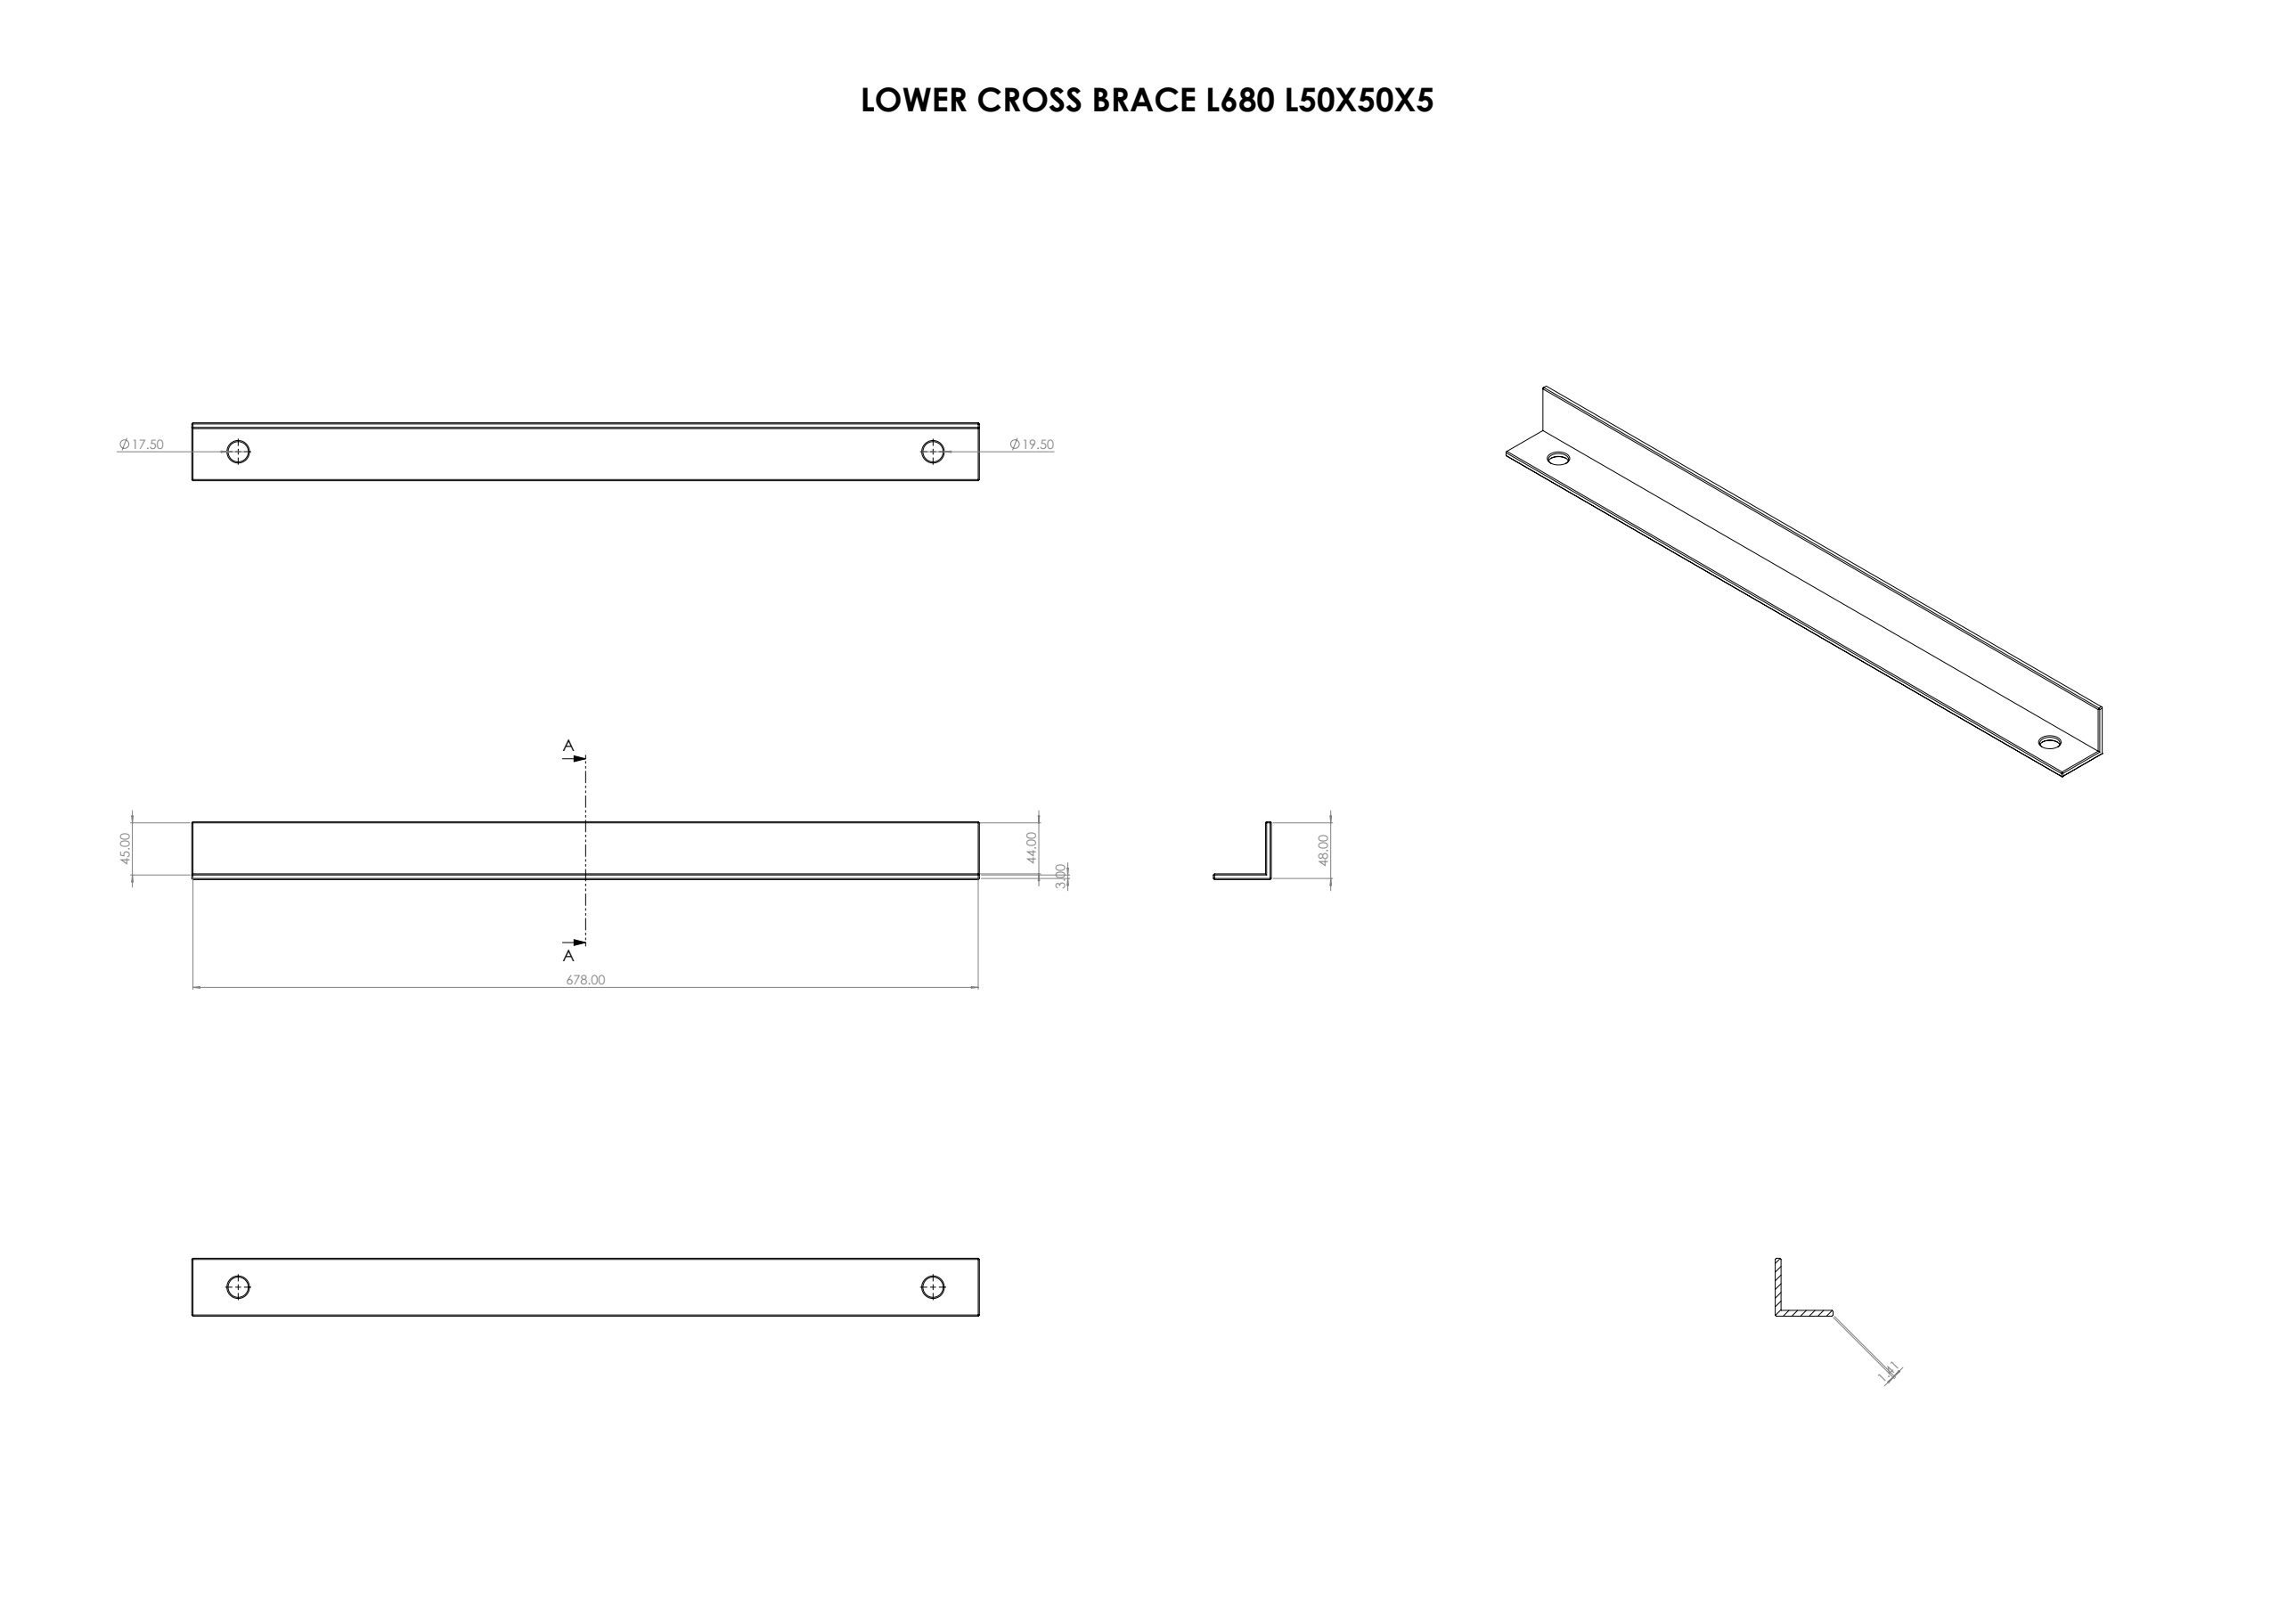
ISO-10303-21;
HEADER;
/* Generated by software containing ST-Developer
 * from STEP Tools, Inc. (www.steptools.com) 
 */

FILE_DESCRIPTION(
/* description */ (''),
/* implementation_level */ '2;1');

FILE_NAME(
/* name */ '08_Lower_Cross_Brace_L680_L50x50x5.step',
/* time_stamp */ '2026-10-20T10:03:03-07:00',
/* author */ (''),
/* organization */ (''),
/* preprocessor_version */ 'ST-DEVELOPER v20.2',
/* originating_system */ 'Autodesk Translation Framework v15.15.0.0',
/* authorisation */ '');

FILE_SCHEMA (('AUTOMOTIVE_DESIGN { 1 0 10303 214 3 1 1 }'));
ENDSEC;

DATA;
#10=MECHANICAL_DESIGN_GEOMETRIC_PRESENTATION_REPRESENTATION('',(#527),#71492);
#385=SHAPE_REPRESENTATION_RELATIONSHIP('SRR','None',#71606,#404);
#404=ADVANCED_BREP_SHAPE_REPRESENTATION('',(#423),#71476);
#423=MANIFOLD_SOLID_BREP('Brace',#28462);
#527=STYLED_ITEM('',(#71873),#423);
#1573=CYLINDRICAL_SURFACE('',#29328,0.875);
#1574=CYLINDRICAL_SURFACE('',#29333,0.875);
#1914=FACE_BOUND('',#5135,.T.);
#1915=FACE_BOUND('',#5136,.T.);
#1916=FACE_BOUND('',#5140,.T.);
#1917=FACE_BOUND('',#5141,.T.);
#2230=CIRCLE('',#29316,0.975000000000001);
#2231=CIRCLE('',#29317,0.975000000000001);
#2232=CIRCLE('',#29321,0.975000000000001);
#2233=CIRCLE('',#29322,0.975000000000001);
#2234=CIRCLE('',#29327,0.875);
#2235=CIRCLE('',#29329,0.875);
#2236=CIRCLE('',#29332,0.875);
#2237=CIRCLE('',#29334,0.875);
#2815=CONICAL_SURFACE('',#29326,0.925000000000001,0.785398163397457);
#2816=CONICAL_SURFACE('',#29330,0.925000000000001,0.785398163397457);
#2817=CONICAL_SURFACE('',#29331,0.925000000000001,0.785398163397457);
#2818=CONICAL_SURFACE('',#29335,0.925000000000001,0.785398163397457);
#3506=FACE_OUTER_BOUND('',#5126,.T.);
#3507=FACE_OUTER_BOUND('',#5127,.T.);
#3508=FACE_OUTER_BOUND('',#5128,.T.);
#3509=FACE_OUTER_BOUND('',#5129,.T.);
#3510=FACE_OUTER_BOUND('',#5130,.T.);
#3511=FACE_OUTER_BOUND('',#5131,.T.);
#3512=FACE_OUTER_BOUND('',#5132,.T.);
#3513=FACE_OUTER_BOUND('',#5133,.T.);
#3514=FACE_OUTER_BOUND('',#5134,.T.);
#3515=FACE_OUTER_BOUND('',#5137,.T.);
#3516=FACE_OUTER_BOUND('',#5138,.T.);
#3517=FACE_OUTER_BOUND('',#5139,.T.);
#3518=FACE_OUTER_BOUND('',#5142,.T.);
#3519=FACE_OUTER_BOUND('',#5143,.T.);
#3520=FACE_OUTER_BOUND('',#5144,.T.);
#3521=FACE_OUTER_BOUND('',#5145,.T.);
#3522=FACE_OUTER_BOUND('',#5146,.T.);
#3523=FACE_OUTER_BOUND('',#5147,.T.);
#3524=FACE_OUTER_BOUND('',#5148,.T.);
#3525=FACE_OUTER_BOUND('',#5149,.T.);
#3526=FACE_OUTER_BOUND('',#5150,.T.);
#3527=FACE_OUTER_BOUND('',#5151,.T.);
#3528=FACE_OUTER_BOUND('',#5152,.T.);
#3529=FACE_OUTER_BOUND('',#5153,.T.);
#3530=FACE_OUTER_BOUND('',#5154,.T.);
#3531=FACE_OUTER_BOUND('',#5155,.T.);
#3532=FACE_OUTER_BOUND('',#5156,.T.);
#3533=FACE_OUTER_BOUND('',#5157,.T.);
#3534=FACE_OUTER_BOUND('',#5158,.T.);
#3535=FACE_OUTER_BOUND('',#5159,.T.);
#3536=FACE_OUTER_BOUND('',#5160,.T.);
#5126=EDGE_LOOP('',(#20811,#20812,#20813,#20814,#20815,#20816));
#5127=EDGE_LOOP('',(#20817,#20818,#20819,#20820,#20821,#20822));
#5128=EDGE_LOOP('',(#20823,#20824,#20825,#20826));
#5129=EDGE_LOOP('',(#20827,#20828,#20829,#20830,#20831,#20832));
#5130=EDGE_LOOP('',(#20833,#20834,#20835,#20836,#20837,#20838));
#5131=EDGE_LOOP('',(#20839,#20840,#20841,#20842,#20843,#20844));
#5132=EDGE_LOOP('',(#20845,#20846,#20847,#20848,#20849,#20850));
#5133=EDGE_LOOP('',(#20851,#20852,#20853,#20854,#20855));
#5134=EDGE_LOOP('',(#20856,#20857,#20858,#20859));
#5135=EDGE_LOOP('',(#20860));
#5136=EDGE_LOOP('',(#20861));
#5137=EDGE_LOOP('',(#20862,#20863,#20864,#20865,#20866,#20867));
#5138=EDGE_LOOP('',(#20868,#20869,#20870,#20871,#20872,#20873));
#5139=EDGE_LOOP('',(#20874,#20875,#20876,#20877));
#5140=EDGE_LOOP('',(#20878));
#5141=EDGE_LOOP('',(#20879));
#5142=EDGE_LOOP('',(#20880,#20881,#20882,#20883,#20884,#20885));
#5143=EDGE_LOOP('',(#20886,#20887,#20888,#20889,#20890,#20891));
#5144=EDGE_LOOP('',(#20892,#20893,#20894,#20895,#20896,#20897));
#5145=EDGE_LOOP('',(#20898,#20899,#20900,#20901));
#5146=EDGE_LOOP('',(#20902,#20903,#20904,#20905));
#5147=EDGE_LOOP('',(#20906,#20907,#20908,#20909));
#5148=EDGE_LOOP('',(#20910,#20911,#20912,#20913));
#5149=EDGE_LOOP('',(#20914,#20915,#20916,#20917));
#5150=EDGE_LOOP('',(#20918,#20919,#20920,#20921));
#5151=EDGE_LOOP('',(#20922,#20923,#20924,#20925,#20926));
#5152=EDGE_LOOP('',(#20927,#20928,#20929,#20930,#20931));
#5153=EDGE_LOOP('',(#20932,#20933,#20934,#20935,#20936,#20937));
#5154=EDGE_LOOP('',(#20938,#20939,#20940,#20941));
#5155=EDGE_LOOP('',(#20942,#20943,#20944,#20945,#20946,#20947));
#5156=EDGE_LOOP('',(#20948,#20949,#20950,#20951,#20952,#20953));
#5157=EDGE_LOOP('',(#20954,#20955,#20956,#20957,#20958));
#5158=EDGE_LOOP('',(#20959,#20960,#20961,#20962));
#5159=EDGE_LOOP('',(#20963,#20964,#20965,#20966,#20967,#20968));
#5160=EDGE_LOOP('',(#20969,#20970,#20971,#20972));
#7329=LINE('',#43368,#9817);
#7330=LINE('',#43370,#9818);
#7331=LINE('',#43372,#9819);
#7332=LINE('',#43374,#9820);
#7333=LINE('',#43376,#9821);
#7334=LINE('',#43377,#9822);
#7335=LINE('',#43380,#9823);
#7336=LINE('',#43382,#9824);
#7337=LINE('',#43384,#9825);
#7338=LINE('',#43386,#9826);
#7339=LINE('',#43387,#9827);
#7340=LINE('',#43390,#9828);
#7341=LINE('',#43391,#9829);
#7342=LINE('',#43394,#9830);
#7343=LINE('',#43396,#9831);
#7344=LINE('',#43398,#9832);
#7345=LINE('',#43399,#9833);
#7346=LINE('',#43402,#9834);
#7347=LINE('',#43404,#9835);
#7348=LINE('',#43405,#9836);
#7349=LINE('',#43409,#9837);
#7350=LINE('',#43411,#9838);
#7351=LINE('',#43413,#9839);
#7352=LINE('',#43415,#9840);
#7353=LINE('',#43417,#9841);
#7354=LINE('',#43418,#9842);
#7355=LINE('',#43421,#9843);
#7356=LINE('',#43423,#9844);
#7357=LINE('',#43425,#9845);
#7358=LINE('',#43427,#9846);
#7359=LINE('',#43428,#9847);
#7360=LINE('',#43431,#9848);
#7361=LINE('',#43433,#9849);
#7362=LINE('',#43434,#9850);
#7363=LINE('',#43437,#9851);
#7364=LINE('',#43438,#9852);
#7365=LINE('',#43446,#9853);
#7366=LINE('',#43448,#9854);
#7367=LINE('',#43450,#9855);
#7368=LINE('',#43452,#9856);
#7369=LINE('',#43454,#9857);
#7370=LINE('',#43455,#9858);
#7371=LINE('',#43458,#9859);
#7372=LINE('',#43459,#9860);
#7373=LINE('',#43461,#9861);
#7374=LINE('',#43462,#9862);
#7375=LINE('',#43465,#9863);
#7376=LINE('',#43466,#9864);
#7377=LINE('',#43473,#9865);
#7378=LINE('',#43475,#9866);
#7379=LINE('',#43477,#9867);
#7380=LINE('',#43478,#9868);
#7381=LINE('',#43481,#9869);
#7382=LINE('',#43482,#9870);
#7383=LINE('',#43484,#9871);
#7384=LINE('',#43486,#9872);
#7385=LINE('',#43487,#9873);
#7386=LINE('',#43490,#9874);
#7387=LINE('',#43495,#9875);
#7388=LINE('',#43497,#9876);
#7389=LINE('',#43500,#9877);
#7390=LINE('',#43505,#9878);
#7391=LINE('',#43507,#9879);
#7392=LINE('',#43510,#9880);
#7393=LINE('',#43511,#9881);
#7394=LINE('',#43513,#9882);
#7395=LINE('',#43514,#9883);
#7396=LINE('',#43516,#9884);
#7397=LINE('',#43517,#9885);
#7398=LINE('',#43521,#9886);
#7399=LINE('',#43522,#9887);
#7400=LINE('',#43524,#9888);
#7401=LINE('',#43525,#9889);
#9817=VECTOR('',#33122,1.);
#9818=VECTOR('',#33123,1.);
#9819=VECTOR('',#33124,1.);
#9820=VECTOR('',#33125,1.);
#9821=VECTOR('',#33126,1.);
#9822=VECTOR('',#33127,1.);
#9823=VECTOR('',#33130,1.);
#9824=VECTOR('',#33131,1.);
#9825=VECTOR('',#33132,1.);
#9826=VECTOR('',#33133,1.);
#9827=VECTOR('',#33134,1.);
#9828=VECTOR('',#33137,1.);
#9829=VECTOR('',#33138,1.);
#9830=VECTOR('',#33141,1.);
#9831=VECTOR('',#33142,1.);
#9832=VECTOR('',#33143,1.);
#9833=VECTOR('',#33144,1.);
#9834=VECTOR('',#33147,1.);
#9835=VECTOR('',#33148,1.);
#9836=VECTOR('',#33149,1.);
#9837=VECTOR('',#33152,1.);
#9838=VECTOR('',#33153,1.);
#9839=VECTOR('',#33154,1.);
#9840=VECTOR('',#33155,1.);
#9841=VECTOR('',#33156,1.);
#9842=VECTOR('',#33157,1.);
#9843=VECTOR('',#33160,1.);
#9844=VECTOR('',#33161,1.);
#9845=VECTOR('',#33162,1.);
#9846=VECTOR('',#33163,1.);
#9847=VECTOR('',#33164,1.);
#9848=VECTOR('',#33167,1.);
#9849=VECTOR('',#33168,1.);
#9850=VECTOR('',#33169,1.);
#9851=VECTOR('',#33172,1.);
#9852=VECTOR('',#33173,1.);
#9853=VECTOR('',#33180,1.);
#9854=VECTOR('',#33181,1.);
#9855=VECTOR('',#33182,1.);
#9856=VECTOR('',#33183,1.);
#9857=VECTOR('',#33184,1.);
#9858=VECTOR('',#33185,1.);
#9859=VECTOR('',#33188,1.);
#9860=VECTOR('',#33189,1.);
#9861=VECTOR('',#33190,1.);
#9862=VECTOR('',#33191,1.);
#9863=VECTOR('',#33194,1.);
#9864=VECTOR('',#33195,1.);
#9865=VECTOR('',#33202,1.);
#9866=VECTOR('',#33203,1.);
#9867=VECTOR('',#33204,1.);
#9868=VECTOR('',#33205,1.);
#9869=VECTOR('',#33208,1.);
#9870=VECTOR('',#33209,1.);
#9871=VECTOR('',#33212,1.);
#9872=VECTOR('',#33213,1.);
#9873=VECTOR('',#33214,1.);
#9874=VECTOR('',#33217,0.925000000000001);
#9875=VECTOR('',#33224,0.875);
#9876=VECTOR('',#33227,0.925000000000001);
#9877=VECTOR('',#33230,0.925000000000001);
#9878=VECTOR('',#33237,0.875);
#9879=VECTOR('',#33240,0.925000000000001);
#9880=VECTOR('',#33243,1.);
#9881=VECTOR('',#33244,1.);
#9882=VECTOR('',#33247,1.);
#9883=VECTOR('',#33248,1.);
#9884=VECTOR('',#33251,1.);
#9885=VECTOR('',#33252,1.);
#9886=VECTOR('',#33259,1.);
#9887=VECTOR('',#33260,1.);
#9888=VECTOR('',#33263,1.);
#9889=VECTOR('',#33264,1.);
#12183=VERTEX_POINT('',#43366);
#12184=VERTEX_POINT('',#43367);
#12185=VERTEX_POINT('',#43369);
#12186=VERTEX_POINT('',#43371);
#12187=VERTEX_POINT('',#43373);
#12188=VERTEX_POINT('',#43375);
#12189=VERTEX_POINT('',#43379);
#12190=VERTEX_POINT('',#43381);
#12191=VERTEX_POINT('',#43383);
#12192=VERTEX_POINT('',#43385);
#12193=VERTEX_POINT('',#43389);
#12194=VERTEX_POINT('',#43393);
#12195=VERTEX_POINT('',#43395);
#12196=VERTEX_POINT('',#43397);
#12197=VERTEX_POINT('',#43401);
#12198=VERTEX_POINT('',#43403);
#12199=VERTEX_POINT('',#43407);
#12200=VERTEX_POINT('',#43408);
#12201=VERTEX_POINT('',#43410);
#12202=VERTEX_POINT('',#43412);
#12203=VERTEX_POINT('',#43414);
#12204=VERTEX_POINT('',#43416);
#12205=VERTEX_POINT('',#43420);
#12206=VERTEX_POINT('',#43422);
#12207=VERTEX_POINT('',#43424);
#12208=VERTEX_POINT('',#43426);
#12209=VERTEX_POINT('',#43430);
#12210=VERTEX_POINT('',#43432);
#12211=VERTEX_POINT('',#43436);
#12212=VERTEX_POINT('',#43439);
#12213=VERTEX_POINT('',#43441);
#12214=VERTEX_POINT('',#43444);
#12215=VERTEX_POINT('',#43445);
#12216=VERTEX_POINT('',#43447);
#12217=VERTEX_POINT('',#43449);
#12218=VERTEX_POINT('',#43451);
#12219=VERTEX_POINT('',#43453);
#12220=VERTEX_POINT('',#43457);
#12221=VERTEX_POINT('',#43460);
#12222=VERTEX_POINT('',#43464);
#12223=VERTEX_POINT('',#43467);
#12224=VERTEX_POINT('',#43469);
#12225=VERTEX_POINT('',#43472);
#12226=VERTEX_POINT('',#43474);
#12227=VERTEX_POINT('',#43476);
#12228=VERTEX_POINT('',#43480);
#12229=VERTEX_POINT('',#43485);
#12230=VERTEX_POINT('',#43489);
#12231=VERTEX_POINT('',#43493);
#12232=VERTEX_POINT('',#43499);
#12233=VERTEX_POINT('',#43503);
#12234=VERTEX_POINT('',#43509);
#15289=EDGE_CURVE('',#12183,#12184,#7329,.T.);
#15290=EDGE_CURVE('',#12184,#12185,#7330,.T.);
#15291=EDGE_CURVE('',#12185,#12186,#7331,.T.);
#15292=EDGE_CURVE('',#12186,#12187,#7332,.T.);
#15293=EDGE_CURVE('',#12187,#12188,#7333,.T.);
#15294=EDGE_CURVE('',#12188,#12183,#7334,.T.);
#15295=EDGE_CURVE('',#12185,#12189,#7335,.T.);
#15296=EDGE_CURVE('',#12190,#12189,#7336,.T.);
#15297=EDGE_CURVE('',#12190,#12191,#7337,.T.);
#15298=EDGE_CURVE('',#12191,#12192,#7338,.T.);
#15299=EDGE_CURVE('',#12192,#12186,#7339,.T.);
#15300=EDGE_CURVE('',#12193,#12184,#7340,.T.);
#15301=EDGE_CURVE('',#12189,#12193,#7341,.T.);
#15302=EDGE_CURVE('',#12194,#12183,#7342,.T.);
#15303=EDGE_CURVE('',#12194,#12195,#7343,.T.);
#15304=EDGE_CURVE('',#12195,#12196,#7344,.T.);
#15305=EDGE_CURVE('',#12193,#12196,#7345,.T.);
#15306=EDGE_CURVE('',#12196,#12197,#7346,.T.);
#15307=EDGE_CURVE('',#12197,#12198,#7347,.T.);
#15308=EDGE_CURVE('',#12198,#12190,#7348,.T.);
#15309=EDGE_CURVE('',#12199,#12200,#7349,.T.);
#15310=EDGE_CURVE('',#12200,#12201,#7350,.T.);
#15311=EDGE_CURVE('',#12201,#12202,#7351,.T.);
#15312=EDGE_CURVE('',#12202,#12203,#7352,.T.);
#15313=EDGE_CURVE('',#12203,#12204,#7353,.T.);
#15314=EDGE_CURVE('',#12204,#12199,#7354,.T.);
#15315=EDGE_CURVE('',#12205,#12202,#7355,.T.);
#15316=EDGE_CURVE('',#12205,#12206,#7356,.T.);
#15317=EDGE_CURVE('',#12206,#12207,#7357,.T.);
#15318=EDGE_CURVE('',#12208,#12207,#7358,.T.);
#15319=EDGE_CURVE('',#12208,#12203,#7359,.T.);
#15320=EDGE_CURVE('',#12201,#12209,#7360,.T.);
#15321=EDGE_CURVE('',#12210,#12209,#7361,.T.);
#15322=EDGE_CURVE('',#12210,#12205,#7362,.T.);
#15323=EDGE_CURVE('',#12211,#12200,#7363,.T.);
#15324=EDGE_CURVE('',#12209,#12211,#7364,.T.);
#15325=EDGE_CURVE('',#12212,#12212,#2230,.T.);
#15326=EDGE_CURVE('',#12213,#12213,#2231,.T.);
#15327=EDGE_CURVE('',#12214,#12215,#7365,.T.);
#15328=EDGE_CURVE('',#12215,#12216,#7366,.T.);
#15329=EDGE_CURVE('',#12216,#12217,#7367,.T.);
#15330=EDGE_CURVE('',#12217,#12218,#7368,.T.);
#15331=EDGE_CURVE('',#12218,#12219,#7369,.T.);
#15332=EDGE_CURVE('',#12219,#12214,#7370,.T.);
#15333=EDGE_CURVE('',#12216,#12220,#7371,.T.);
#15334=EDGE_CURVE('',#12207,#12220,#7372,.T.);
#15335=EDGE_CURVE('',#12206,#12221,#7373,.T.);
#15336=EDGE_CURVE('',#12221,#12217,#7374,.T.);
#15337=EDGE_CURVE('',#12222,#12215,#7375,.T.);
#15338=EDGE_CURVE('',#12220,#12222,#7376,.T.);
#15339=EDGE_CURVE('',#12223,#12223,#2232,.T.);
#15340=EDGE_CURVE('',#12224,#12224,#2233,.T.);
#15341=EDGE_CURVE('',#12225,#12214,#7377,.T.);
#15342=EDGE_CURVE('',#12225,#12226,#7378,.T.);
#15343=EDGE_CURVE('',#12226,#12227,#7379,.T.);
#15344=EDGE_CURVE('',#12222,#12227,#7380,.T.);
#15345=EDGE_CURVE('',#12227,#12228,#7381,.T.);
#15346=EDGE_CURVE('',#12228,#12208,#7382,.T.);
#15347=EDGE_CURVE('',#12204,#12228,#7383,.T.);
#15348=EDGE_CURVE('',#12226,#12229,#7384,.T.);
#15349=EDGE_CURVE('',#12229,#12199,#7385,.T.);
#15350=EDGE_CURVE('',#12212,#12230,#7386,.T.);
#15351=EDGE_CURVE('',#12230,#12230,#2234,.T.);
#15352=EDGE_CURVE('',#12231,#12231,#2235,.T.);
#15353=EDGE_CURVE('',#12231,#12230,#7387,.T.);
#15354=EDGE_CURVE('',#12224,#12231,#7388,.T.);
#15355=EDGE_CURVE('',#12213,#12232,#7389,.T.);
#15356=EDGE_CURVE('',#12232,#12232,#2236,.T.);
#15357=EDGE_CURVE('',#12233,#12233,#2237,.T.);
#15358=EDGE_CURVE('',#12233,#12232,#7390,.T.);
#15359=EDGE_CURVE('',#12223,#12233,#7391,.T.);
#15360=EDGE_CURVE('',#12229,#12234,#7392,.T.);
#15361=EDGE_CURVE('',#12234,#12211,#7393,.T.);
#15362=EDGE_CURVE('',#12188,#12211,#7394,.T.);
#15363=EDGE_CURVE('',#12234,#12194,#7395,.T.);
#15364=EDGE_CURVE('',#12195,#12225,#7396,.T.);
#15365=EDGE_CURVE('',#12219,#12197,#7397,.T.);
#15366=EDGE_CURVE('',#12198,#12218,#7398,.T.);
#15367=EDGE_CURVE('',#12221,#12191,#7399,.T.);
#15368=EDGE_CURVE('',#12192,#12210,#7400,.T.);
#15369=EDGE_CURVE('',#12209,#12187,#7401,.T.);
#20811=ORIENTED_EDGE('',*,*,#15289,.T.);
#20812=ORIENTED_EDGE('',*,*,#15290,.T.);
#20813=ORIENTED_EDGE('',*,*,#15291,.T.);
#20814=ORIENTED_EDGE('',*,*,#15292,.T.);
#20815=ORIENTED_EDGE('',*,*,#15293,.T.);
#20816=ORIENTED_EDGE('',*,*,#15294,.T.);
#20817=ORIENTED_EDGE('',*,*,#15291,.F.);
#20818=ORIENTED_EDGE('',*,*,#15295,.T.);
#20819=ORIENTED_EDGE('',*,*,#15296,.F.);
#20820=ORIENTED_EDGE('',*,*,#15297,.T.);
#20821=ORIENTED_EDGE('',*,*,#15298,.T.);
#20822=ORIENTED_EDGE('',*,*,#15299,.T.);
#20823=ORIENTED_EDGE('',*,*,#15290,.F.);
#20824=ORIENTED_EDGE('',*,*,#15300,.F.);
#20825=ORIENTED_EDGE('',*,*,#15301,.F.);
#20826=ORIENTED_EDGE('',*,*,#15295,.F.);
#20827=ORIENTED_EDGE('',*,*,#15289,.F.);
#20828=ORIENTED_EDGE('',*,*,#15302,.F.);
#20829=ORIENTED_EDGE('',*,*,#15303,.T.);
#20830=ORIENTED_EDGE('',*,*,#15304,.T.);
#20831=ORIENTED_EDGE('',*,*,#15305,.F.);
#20832=ORIENTED_EDGE('',*,*,#15300,.T.);
#20833=ORIENTED_EDGE('',*,*,#15306,.T.);
#20834=ORIENTED_EDGE('',*,*,#15307,.T.);
#20835=ORIENTED_EDGE('',*,*,#15308,.T.);
#20836=ORIENTED_EDGE('',*,*,#15296,.T.);
#20837=ORIENTED_EDGE('',*,*,#15301,.T.);
#20838=ORIENTED_EDGE('',*,*,#15305,.T.);
#20839=ORIENTED_EDGE('',*,*,#15309,.T.);
#20840=ORIENTED_EDGE('',*,*,#15310,.T.);
#20841=ORIENTED_EDGE('',*,*,#15311,.T.);
#20842=ORIENTED_EDGE('',*,*,#15312,.T.);
#20843=ORIENTED_EDGE('',*,*,#15313,.T.);
#20844=ORIENTED_EDGE('',*,*,#15314,.T.);
#20845=ORIENTED_EDGE('',*,*,#15312,.F.);
#20846=ORIENTED_EDGE('',*,*,#15315,.F.);
#20847=ORIENTED_EDGE('',*,*,#15316,.T.);
#20848=ORIENTED_EDGE('',*,*,#15317,.T.);
#20849=ORIENTED_EDGE('',*,*,#15318,.F.);
#20850=ORIENTED_EDGE('',*,*,#15319,.T.);
#20851=ORIENTED_EDGE('',*,*,#15311,.F.);
#20852=ORIENTED_EDGE('',*,*,#15320,.T.);
#20853=ORIENTED_EDGE('',*,*,#15321,.F.);
#20854=ORIENTED_EDGE('',*,*,#15322,.T.);
#20855=ORIENTED_EDGE('',*,*,#15315,.T.);
#20856=ORIENTED_EDGE('',*,*,#15310,.F.);
#20857=ORIENTED_EDGE('',*,*,#15323,.F.);
#20858=ORIENTED_EDGE('',*,*,#15324,.F.);
#20859=ORIENTED_EDGE('',*,*,#15320,.F.);
#20860=ORIENTED_EDGE('',*,*,#15325,.F.);
#20861=ORIENTED_EDGE('',*,*,#15326,.F.);
#20862=ORIENTED_EDGE('',*,*,#15327,.T.);
#20863=ORIENTED_EDGE('',*,*,#15328,.T.);
#20864=ORIENTED_EDGE('',*,*,#15329,.T.);
#20865=ORIENTED_EDGE('',*,*,#15330,.T.);
#20866=ORIENTED_EDGE('',*,*,#15331,.T.);
#20867=ORIENTED_EDGE('',*,*,#15332,.T.);
#20868=ORIENTED_EDGE('',*,*,#15329,.F.);
#20869=ORIENTED_EDGE('',*,*,#15333,.T.);
#20870=ORIENTED_EDGE('',*,*,#15334,.F.);
#20871=ORIENTED_EDGE('',*,*,#15317,.F.);
#20872=ORIENTED_EDGE('',*,*,#15335,.T.);
#20873=ORIENTED_EDGE('',*,*,#15336,.T.);
#20874=ORIENTED_EDGE('',*,*,#15328,.F.);
#20875=ORIENTED_EDGE('',*,*,#15337,.F.);
#20876=ORIENTED_EDGE('',*,*,#15338,.F.);
#20877=ORIENTED_EDGE('',*,*,#15333,.F.);
#20878=ORIENTED_EDGE('',*,*,#15339,.F.);
#20879=ORIENTED_EDGE('',*,*,#15340,.F.);
#20880=ORIENTED_EDGE('',*,*,#15327,.F.);
#20881=ORIENTED_EDGE('',*,*,#15341,.F.);
#20882=ORIENTED_EDGE('',*,*,#15342,.T.);
#20883=ORIENTED_EDGE('',*,*,#15343,.T.);
#20884=ORIENTED_EDGE('',*,*,#15344,.F.);
#20885=ORIENTED_EDGE('',*,*,#15337,.T.);
#20886=ORIENTED_EDGE('',*,*,#15345,.T.);
#20887=ORIENTED_EDGE('',*,*,#15346,.T.);
#20888=ORIENTED_EDGE('',*,*,#15318,.T.);
#20889=ORIENTED_EDGE('',*,*,#15334,.T.);
#20890=ORIENTED_EDGE('',*,*,#15338,.T.);
#20891=ORIENTED_EDGE('',*,*,#15344,.T.);
#20892=ORIENTED_EDGE('',*,*,#15314,.F.);
#20893=ORIENTED_EDGE('',*,*,#15347,.T.);
#20894=ORIENTED_EDGE('',*,*,#15345,.F.);
#20895=ORIENTED_EDGE('',*,*,#15343,.F.);
#20896=ORIENTED_EDGE('',*,*,#15348,.T.);
#20897=ORIENTED_EDGE('',*,*,#15349,.T.);
#20898=ORIENTED_EDGE('',*,*,#15325,.T.);
#20899=ORIENTED_EDGE('',*,*,#15350,.T.);
#20900=ORIENTED_EDGE('',*,*,#15351,.T.);
#20901=ORIENTED_EDGE('',*,*,#15350,.F.);
#20902=ORIENTED_EDGE('',*,*,#15352,.F.);
#20903=ORIENTED_EDGE('',*,*,#15353,.T.);
#20904=ORIENTED_EDGE('',*,*,#15351,.F.);
#20905=ORIENTED_EDGE('',*,*,#15353,.F.);
#20906=ORIENTED_EDGE('',*,*,#15340,.T.);
#20907=ORIENTED_EDGE('',*,*,#15354,.T.);
#20908=ORIENTED_EDGE('',*,*,#15352,.T.);
#20909=ORIENTED_EDGE('',*,*,#15354,.F.);
#20910=ORIENTED_EDGE('',*,*,#15326,.T.);
#20911=ORIENTED_EDGE('',*,*,#15355,.T.);
#20912=ORIENTED_EDGE('',*,*,#15356,.T.);
#20913=ORIENTED_EDGE('',*,*,#15355,.F.);
#20914=ORIENTED_EDGE('',*,*,#15357,.F.);
#20915=ORIENTED_EDGE('',*,*,#15358,.T.);
#20916=ORIENTED_EDGE('',*,*,#15356,.F.);
#20917=ORIENTED_EDGE('',*,*,#15358,.F.);
#20918=ORIENTED_EDGE('',*,*,#15339,.T.);
#20919=ORIENTED_EDGE('',*,*,#15359,.T.);
#20920=ORIENTED_EDGE('',*,*,#15357,.T.);
#20921=ORIENTED_EDGE('',*,*,#15359,.F.);
#20922=ORIENTED_EDGE('',*,*,#15309,.F.);
#20923=ORIENTED_EDGE('',*,*,#15349,.F.);
#20924=ORIENTED_EDGE('',*,*,#15360,.T.);
#20925=ORIENTED_EDGE('',*,*,#15361,.T.);
#20926=ORIENTED_EDGE('',*,*,#15323,.T.);
#20927=ORIENTED_EDGE('',*,*,#15294,.F.);
#20928=ORIENTED_EDGE('',*,*,#15362,.T.);
#20929=ORIENTED_EDGE('',*,*,#15361,.F.);
#20930=ORIENTED_EDGE('',*,*,#15363,.T.);
#20931=ORIENTED_EDGE('',*,*,#15302,.T.);
#20932=ORIENTED_EDGE('',*,*,#15306,.F.);
#20933=ORIENTED_EDGE('',*,*,#15304,.F.);
#20934=ORIENTED_EDGE('',*,*,#15364,.T.);
#20935=ORIENTED_EDGE('',*,*,#15341,.T.);
#20936=ORIENTED_EDGE('',*,*,#15332,.F.);
#20937=ORIENTED_EDGE('',*,*,#15365,.T.);
#20938=ORIENTED_EDGE('',*,*,#15313,.F.);
#20939=ORIENTED_EDGE('',*,*,#15319,.F.);
#20940=ORIENTED_EDGE('',*,*,#15346,.F.);
#20941=ORIENTED_EDGE('',*,*,#15347,.F.);
#20942=ORIENTED_EDGE('',*,*,#15360,.F.);
#20943=ORIENTED_EDGE('',*,*,#15348,.F.);
#20944=ORIENTED_EDGE('',*,*,#15342,.F.);
#20945=ORIENTED_EDGE('',*,*,#15364,.F.);
#20946=ORIENTED_EDGE('',*,*,#15303,.F.);
#20947=ORIENTED_EDGE('',*,*,#15363,.F.);
#20948=ORIENTED_EDGE('',*,*,#15308,.F.);
#20949=ORIENTED_EDGE('',*,*,#15366,.T.);
#20950=ORIENTED_EDGE('',*,*,#15330,.F.);
#20951=ORIENTED_EDGE('',*,*,#15336,.F.);
#20952=ORIENTED_EDGE('',*,*,#15367,.T.);
#20953=ORIENTED_EDGE('',*,*,#15297,.F.);
#20954=ORIENTED_EDGE('',*,*,#15292,.F.);
#20955=ORIENTED_EDGE('',*,*,#15299,.F.);
#20956=ORIENTED_EDGE('',*,*,#15368,.T.);
#20957=ORIENTED_EDGE('',*,*,#15321,.T.);
#20958=ORIENTED_EDGE('',*,*,#15369,.T.);
#20959=ORIENTED_EDGE('',*,*,#15307,.F.);
#20960=ORIENTED_EDGE('',*,*,#15365,.F.);
#20961=ORIENTED_EDGE('',*,*,#15331,.F.);
#20962=ORIENTED_EDGE('',*,*,#15366,.F.);
#20963=ORIENTED_EDGE('',*,*,#15298,.F.);
#20964=ORIENTED_EDGE('',*,*,#15367,.F.);
#20965=ORIENTED_EDGE('',*,*,#15335,.F.);
#20966=ORIENTED_EDGE('',*,*,#15316,.F.);
#20967=ORIENTED_EDGE('',*,*,#15322,.F.);
#20968=ORIENTED_EDGE('',*,*,#15368,.F.);
#20969=ORIENTED_EDGE('',*,*,#15293,.F.);
#20970=ORIENTED_EDGE('',*,*,#15369,.F.);
#20971=ORIENTED_EDGE('',*,*,#15324,.T.);
#20972=ORIENTED_EDGE('',*,*,#15362,.F.);
#26375=PLANE('',#29307);
#26376=PLANE('',#29308);
#26377=PLANE('',#29309);
#26378=PLANE('',#29310);
#26379=PLANE('',#29311);
#26380=PLANE('',#29312);
#26381=PLANE('',#29313);
#26382=PLANE('',#29314);
#26383=PLANE('',#29315);
#26384=PLANE('',#29318);
#26385=PLANE('',#29319);
#26386=PLANE('',#29320);
#26387=PLANE('',#29323);
#26388=PLANE('',#29324);
#26389=PLANE('',#29325);
#26390=PLANE('',#29336);
#26391=PLANE('',#29337);
#26392=PLANE('',#29338);
#26393=PLANE('',#29339);
#26394=PLANE('',#29340);
#26395=PLANE('',#29341);
#26396=PLANE('',#29342);
#26397=PLANE('',#29343);
#26398=PLANE('',#29344);
#26399=PLANE('',#29345);
#27414=ADVANCED_FACE('',(#3506),#26375,.T.);
#27415=ADVANCED_FACE('',(#3507),#26376,.T.);
#27416=ADVANCED_FACE('',(#3508),#26377,.T.);
#27417=ADVANCED_FACE('',(#3509),#26378,.T.);
#27418=ADVANCED_FACE('',(#3510),#26379,.T.);
#27419=ADVANCED_FACE('',(#3511),#26380,.T.);
#27420=ADVANCED_FACE('',(#3512),#26381,.T.);
#27421=ADVANCED_FACE('',(#3513),#26382,.T.);
#27422=ADVANCED_FACE('',(#3514,#1914,#1915),#26383,.T.);
#27423=ADVANCED_FACE('',(#3515),#26384,.T.);
#27424=ADVANCED_FACE('',(#3516),#26385,.T.);
#27425=ADVANCED_FACE('',(#3517,#1916,#1917),#26386,.T.);
#27426=ADVANCED_FACE('',(#3518),#26387,.T.);
#27427=ADVANCED_FACE('',(#3519),#26388,.T.);
#27428=ADVANCED_FACE('',(#3520),#26389,.T.);
#27429=ADVANCED_FACE('',(#3521),#2815,.F.);
#27430=ADVANCED_FACE('',(#3522),#1573,.F.);
#27431=ADVANCED_FACE('',(#3523),#2816,.F.);
#27432=ADVANCED_FACE('',(#3524),#2817,.F.);
#27433=ADVANCED_FACE('',(#3525),#1574,.F.);
#27434=ADVANCED_FACE('',(#3526),#2818,.F.);
#27435=ADVANCED_FACE('',(#3527),#26390,.T.);
#27436=ADVANCED_FACE('',(#3528),#26391,.T.);
#27437=ADVANCED_FACE('',(#3529),#26392,.T.);
#27438=ADVANCED_FACE('',(#3530),#26393,.T.);
#27439=ADVANCED_FACE('',(#3531),#26394,.T.);
#27440=ADVANCED_FACE('',(#3532),#26395,.T.);
#27441=ADVANCED_FACE('',(#3533),#26396,.T.);
#27442=ADVANCED_FACE('',(#3534),#26397,.T.);
#27443=ADVANCED_FACE('',(#3535),#26398,.F.);
#27444=ADVANCED_FACE('',(#3536),#26399,.T.);
#28462=CLOSED_SHELL('',(#27414,#27415,#27416,#27417,#27418,#27419,#27420,
#27421,#27422,#27423,#27424,#27425,#27426,#27427,#27428,#27429,#27430,#27431,
#27432,#27433,#27434,#27435,#27436,#27437,#27438,#27439,#27440,#27441,#27442,
#27443,#27444));
#29306=AXIS2_PLACEMENT_3D('',#43364,#33118,#33119);
#29307=AXIS2_PLACEMENT_3D('',#43365,#33120,#33121);
#29308=AXIS2_PLACEMENT_3D('',#43378,#33128,#33129);
#29309=AXIS2_PLACEMENT_3D('',#43388,#33135,#33136);
#29310=AXIS2_PLACEMENT_3D('',#43392,#33139,#33140);
#29311=AXIS2_PLACEMENT_3D('',#43400,#33145,#33146);
#29312=AXIS2_PLACEMENT_3D('',#43406,#33150,#33151);
#29313=AXIS2_PLACEMENT_3D('',#43419,#33158,#33159);
#29314=AXIS2_PLACEMENT_3D('',#43429,#33165,#33166);
#29315=AXIS2_PLACEMENT_3D('',#43435,#33170,#33171);
#29316=AXIS2_PLACEMENT_3D('',#43440,#33174,#33175);
#29317=AXIS2_PLACEMENT_3D('',#43442,#33176,#33177);
#29318=AXIS2_PLACEMENT_3D('',#43443,#33178,#33179);
#29319=AXIS2_PLACEMENT_3D('',#43456,#33186,#33187);
#29320=AXIS2_PLACEMENT_3D('',#43463,#33192,#33193);
#29321=AXIS2_PLACEMENT_3D('',#43468,#33196,#33197);
#29322=AXIS2_PLACEMENT_3D('',#43470,#33198,#33199);
#29323=AXIS2_PLACEMENT_3D('',#43471,#33200,#33201);
#29324=AXIS2_PLACEMENT_3D('',#43479,#33206,#33207);
#29325=AXIS2_PLACEMENT_3D('',#43483,#33210,#33211);
#29326=AXIS2_PLACEMENT_3D('',#43488,#33215,#33216);
#29327=AXIS2_PLACEMENT_3D('',#43491,#33218,#33219);
#29328=AXIS2_PLACEMENT_3D('',#43492,#33220,#33221);
#29329=AXIS2_PLACEMENT_3D('',#43494,#33222,#33223);
#29330=AXIS2_PLACEMENT_3D('',#43496,#33225,#33226);
#29331=AXIS2_PLACEMENT_3D('',#43498,#33228,#33229);
#29332=AXIS2_PLACEMENT_3D('',#43501,#33231,#33232);
#29333=AXIS2_PLACEMENT_3D('',#43502,#33233,#33234);
#29334=AXIS2_PLACEMENT_3D('',#43504,#33235,#33236);
#29335=AXIS2_PLACEMENT_3D('',#43506,#33238,#33239);
#29336=AXIS2_PLACEMENT_3D('',#43508,#33241,#33242);
#29337=AXIS2_PLACEMENT_3D('',#43512,#33245,#33246);
#29338=AXIS2_PLACEMENT_3D('',#43515,#33249,#33250);
#29339=AXIS2_PLACEMENT_3D('',#43518,#33253,#33254);
#29340=AXIS2_PLACEMENT_3D('',#43519,#33255,#33256);
#29341=AXIS2_PLACEMENT_3D('',#43520,#33257,#33258);
#29342=AXIS2_PLACEMENT_3D('',#43523,#33261,#33262);
#29343=AXIS2_PLACEMENT_3D('',#43526,#33265,#33266);
#29344=AXIS2_PLACEMENT_3D('',#43527,#33267,#33268);
#29345=AXIS2_PLACEMENT_3D('',#43528,#33269,#33270);
#33118=DIRECTION('axis',(0.,0.,1.));
#33119=DIRECTION('refdir',(1.,0.,0.));
#33120=DIRECTION('center_axis',(0.,0.707106781186548,0.707106781186548));
#33121=DIRECTION('ref_axis',(1.,0.,0.));
#33122=DIRECTION('',(-0.577350269189605,0.577350269189636,-0.577350269189636));
#33123=DIRECTION('',(-1.,0.,0.));
#33124=DIRECTION('',(-0.577350269189605,-0.577350269189636,0.577350269189636));
#33125=DIRECTION('',(0.577350269189598,-0.577350269189639,0.577350269189639));
#33126=DIRECTION('',(1.,0.,0.));
#33127=DIRECTION('',(0.577350269189598,0.577350269189639,-0.577350269189639));
#33128=DIRECTION('center_axis',(-0.707106781186566,0.707106781186529,0.));
#33129=DIRECTION('ref_axis',(0.,0.,1.));
#33130=DIRECTION('',(0.,0.,-1.));
#33131=DIRECTION('',(0.577350269189602,0.577350269189633,0.577350269189643));
#33132=DIRECTION('',(-0.577350269189602,-0.577350269189633,0.577350269189643));
#33133=DIRECTION('',(0.,0.,1.));
#33134=DIRECTION('',(0.577350269189602,0.577350269189633,0.577350269189643));
#33135=DIRECTION('center_axis',(0.,1.,0.));
#33136=DIRECTION('ref_axis',(0.,0.,1.));
#33137=DIRECTION('',(0.,0.,1.));
#33138=DIRECTION('',(1.,0.,0.));
#33139=DIRECTION('center_axis',(0.707106781186566,0.707106781186529,0.));
#33140=DIRECTION('ref_axis',(0.,0.,-1.));
#33141=DIRECTION('',(-0.577350269189602,0.577350269189633,0.577350269189643));
#33142=DIRECTION('',(0.,0.,-1.));
#33143=DIRECTION('',(-0.577350269189602,0.577350269189633,-0.577350269189643));
#33144=DIRECTION('',(0.577350269189602,-0.577350269189633,-0.577350269189643));
#33145=DIRECTION('center_axis',(0.,0.707106781186554,-0.707106781186541));
#33146=DIRECTION('ref_axis',(-1.,0.,0.));
#33147=DIRECTION('',(-0.577350269189602,-0.577350269189633,-0.577350269189643));
#33148=DIRECTION('',(-1.,0.,0.));
#33149=DIRECTION('',(-0.577350269189602,0.577350269189633,0.577350269189643));
#33150=DIRECTION('center_axis',(0.,0.707106781186554,0.707106781186541));
#33151=DIRECTION('ref_axis',(1.,0.,0.));
#33152=DIRECTION('',(-0.577350269189602,0.577350269189633,-0.577350269189643));
#33153=DIRECTION('',(-1.,0.,0.));
#33154=DIRECTION('',(-0.577350269189602,-0.577350269189633,0.577350269189643));
#33155=DIRECTION('',(0.577350269189602,-0.577350269189633,0.577350269189643));
#33156=DIRECTION('',(1.,0.,0.));
#33157=DIRECTION('',(0.577350269189602,0.577350269189633,-0.577350269189643));
#33158=DIRECTION('center_axis',(-0.707106781186573,0.,0.707106781186522));
#33159=DIRECTION('ref_axis',(0.707106781186522,0.,0.707106781186573));
#33160=DIRECTION('',(0.577350269189602,0.577350269189633,0.577350269189643));
#33161=DIRECTION('',(0.,-1.,0.));
#33162=DIRECTION('',(0.577350269189602,-0.577350269189633,0.577350269189643));
#33163=DIRECTION('',(-0.577350269189588,-0.57735026918966,-0.577350269189629));
#33164=DIRECTION('',(0.,1.,0.));
#33165=DIRECTION('center_axis',(-0.707106781186566,0.707106781186529,0.));
#33166=DIRECTION('ref_axis',(0.,0.,1.));
#33167=DIRECTION('',(0.,0.,-1.));
#33168=DIRECTION('',(0.577350269189602,0.577350269189633,0.577350269189643));
#33169=DIRECTION('',(0.,0.,1.));
#33170=DIRECTION('center_axis',(0.,1.,0.));
#33171=DIRECTION('ref_axis',(0.,0.,1.));
#33172=DIRECTION('',(0.,0.,1.));
#33173=DIRECTION('',(1.,0.,0.));
#33174=DIRECTION('center_axis',(0.,1.,0.));
#33175=DIRECTION('ref_axis',(1.,0.,0.));
#33176=DIRECTION('center_axis',(0.,1.,0.));
#33177=DIRECTION('ref_axis',(1.,0.,0.));
#33178=DIRECTION('center_axis',(0.,-0.707106781186554,-0.707106781186541));
#33179=DIRECTION('ref_axis',(-1.,0.,0.));
#33180=DIRECTION('',(-0.577350269189602,-0.577350269189633,0.577350269189643));
#33181=DIRECTION('',(-1.,0.,0.));
#33182=DIRECTION('',(-0.577350269189602,0.577350269189633,-0.577350269189643));
#33183=DIRECTION('',(0.577350269189602,0.577350269189633,-0.577350269189643));
#33184=DIRECTION('',(1.,0.,0.));
#33185=DIRECTION('',(0.577350269189602,-0.577350269189633,0.577350269189643));
#33186=DIRECTION('center_axis',(-0.707106781186566,-0.707106781186529,0.));
#33187=DIRECTION('ref_axis',(0.,0.,1.));
#33188=DIRECTION('',(0.,0.,1.));
#33189=DIRECTION('',(0.577350269189616,-0.577350269189646,-0.577350269189616));
#33190=DIRECTION('',(0.,0.,-1.));
#33191=DIRECTION('',(0.577350269189602,-0.577350269189633,-0.577350269189643));
#33192=DIRECTION('center_axis',(0.,-1.,0.));
#33193=DIRECTION('ref_axis',(0.,0.,-1.));
#33194=DIRECTION('',(0.,0.,-1.));
#33195=DIRECTION('',(1.,0.,0.));
#33196=DIRECTION('center_axis',(0.,-1.,0.));
#33197=DIRECTION('ref_axis',(1.,0.,0.));
#33198=DIRECTION('center_axis',(0.,-1.,0.));
#33199=DIRECTION('ref_axis',(1.,0.,0.));
#33200=DIRECTION('center_axis',(0.707106781186566,-0.707106781186529,0.));
#33201=DIRECTION('ref_axis',(0.,0.,-1.));
#33202=DIRECTION('',(-0.577350269189602,-0.577350269189633,-0.577350269189643));
#33203=DIRECTION('',(0.,0.,1.));
#33204=DIRECTION('',(-0.577350269189602,-0.577350269189633,0.577350269189643));
#33205=DIRECTION('',(0.577350269189616,0.577350269189646,0.577350269189616));
#33206=DIRECTION('center_axis',(0.,-0.707106781186529,0.707106781186566));
#33207=DIRECTION('ref_axis',(1.,0.,0.));
#33208=DIRECTION('',(-0.577350269189588,0.57735026918966,0.577350269189629));
#33209=DIRECTION('',(-1.,0.,0.));
#33210=DIRECTION('center_axis',(0.707106781186573,0.,0.707106781186522));
#33211=DIRECTION('ref_axis',(0.707106781186522,0.,-0.707106781186573));
#33212=DIRECTION('',(0.,-1.,0.));
#33213=DIRECTION('',(0.,1.,0.));
#33214=DIRECTION('',(-0.577350269189602,0.577350269189633,0.577350269189643));
#33215=DIRECTION('center_axis',(0.,1.,0.));
#33216=DIRECTION('ref_axis',(1.,0.,0.));
#33217=DIRECTION('',(0.707106781186554,-0.707106781186541,-8.65956056235501E-17));
#33218=DIRECTION('center_axis',(0.,-1.,0.));
#33219=DIRECTION('ref_axis',(1.,0.,0.));
#33220=DIRECTION('center_axis',(0.,1.,0.));
#33221=DIRECTION('ref_axis',(1.,0.,0.));
#33222=DIRECTION('center_axis',(0.,1.,0.));
#33223=DIRECTION('ref_axis',(1.,0.,0.));
#33224=DIRECTION('',(0.,1.,0.));
#33225=DIRECTION('center_axis',(0.,-1.,0.));
#33226=DIRECTION('ref_axis',(1.,0.,0.));
#33227=DIRECTION('',(0.707106781186554,0.707106781186541,8.65956056235501E-17));
#33228=DIRECTION('center_axis',(0.,1.,0.));
#33229=DIRECTION('ref_axis',(1.,0.,0.));
#33230=DIRECTION('',(0.707106781186554,-0.707106781186541,-8.65956056235501E-17));
#33231=DIRECTION('center_axis',(0.,-1.,0.));
#33232=DIRECTION('ref_axis',(1.,0.,0.));
#33233=DIRECTION('center_axis',(0.,1.,0.));
#33234=DIRECTION('ref_axis',(1.,0.,0.));
#33235=DIRECTION('center_axis',(0.,1.,0.));
#33236=DIRECTION('ref_axis',(1.,0.,0.));
#33237=DIRECTION('',(0.,1.,0.));
#33238=DIRECTION('center_axis',(0.,-1.,0.));
#33239=DIRECTION('ref_axis',(1.,0.,0.));
#33240=DIRECTION('',(0.707106781186554,0.707106781186541,8.65956056235501E-17));
#33241=DIRECTION('center_axis',(0.707106781186566,0.707106781186529,0.));
#33242=DIRECTION('ref_axis',(0.,0.,-1.));
#33243=DIRECTION('',(0.,0.,-1.));
#33244=DIRECTION('',(-0.577350269189602,0.577350269189633,0.577350269189643));
#33245=DIRECTION('center_axis',(0.707106781186573,0.,0.707106781186522));
#33246=DIRECTION('ref_axis',(0.707106781186522,0.,-0.707106781186573));
#33247=DIRECTION('',(0.,-1.,0.));
#33248=DIRECTION('',(0.,1.,0.));
#33249=DIRECTION('center_axis',(0.707106781186573,0.,-0.707106781186522));
#33250=DIRECTION('ref_axis',(-0.707106781186522,0.,-0.707106781186573));
#33251=DIRECTION('',(0.,-1.,0.));
#33252=DIRECTION('',(0.,1.,0.));
#33253=DIRECTION('center_axis',(0.,0.,1.));
#33254=DIRECTION('ref_axis',(0.,-1.,0.));
#33255=DIRECTION('center_axis',(1.,0.,0.));
#33256=DIRECTION('ref_axis',(0.,0.,-1.));
#33257=DIRECTION('center_axis',(-0.707106781186573,0.,-0.707106781186522));
#33258=DIRECTION('ref_axis',(-0.707106781186522,0.,0.707106781186573));
#33259=DIRECTION('',(0.,-1.,0.));
#33260=DIRECTION('',(0.,1.,0.));
#33261=DIRECTION('center_axis',(-0.707106781186573,0.,0.707106781186522));
#33262=DIRECTION('ref_axis',(0.707106781186522,0.,0.707106781186573));
#33263=DIRECTION('',(0.,-1.,0.));
#33264=DIRECTION('',(0.,1.,0.));
#33265=DIRECTION('center_axis',(0.,0.,-1.));
#33266=DIRECTION('ref_axis',(0.,1.,0.));
#33267=DIRECTION('center_axis',(1.,0.,0.));
#33268=DIRECTION('ref_axis',(0.,0.,-1.));
#33269=DIRECTION('center_axis',(0.,0.,1.));
#33270=DIRECTION('ref_axis',(0.,-1.,0.));
#43364=CARTESIAN_POINT('',(0.,0.,0.));
#43365=CARTESIAN_POINT('Origin',(-34.,8.95,31.45));
#43366=CARTESIAN_POINT('',(33.95,8.95,31.45));
#43367=CARTESIAN_POINT('',(33.9,9.,31.4));
#43368=CARTESIAN_POINT('',(22.7583333333341,20.1416666666665,20.2583333333335));
#43369=CARTESIAN_POINT('',(-33.9,9.,31.4));
#43370=CARTESIAN_POINT('',(-34.,9.,31.4));
#43371=CARTESIAN_POINT('',(-33.95,8.95,31.45));
#43372=CARTESIAN_POINT('',(-34.0916666666667,8.80833333333333,31.5916666666667));
#43373=CARTESIAN_POINT('',(-33.9,8.9,31.5));
#43374=CARTESIAN_POINT('',(-33.7583333333333,8.75833333333332,31.6416666666667));
#43375=CARTESIAN_POINT('',(33.9,8.9,31.5));
#43376=CARTESIAN_POINT('',(-34.,8.9,31.5));
#43377=CARTESIAN_POINT('',(22.4250000000011,-2.57499999999974,42.9749999999997));
#43378=CARTESIAN_POINT('Origin',(-33.95,8.95,32.25));
#43379=CARTESIAN_POINT('',(-33.9,9.,31.1));
#43380=CARTESIAN_POINT('',(-33.9,9.,32.25));
#43381=CARTESIAN_POINT('',(-33.95,8.95,31.05));
#43382=CARTESIAN_POINT('',(-33.7583333333333,9.14166666666667,31.2416666666667));
#43383=CARTESIAN_POINT('',(-34.,8.9,31.1));
#43384=CARTESIAN_POINT('',(-33.9,9.,31.));
#43385=CARTESIAN_POINT('',(-34.,8.9,31.4));
#43386=CARTESIAN_POINT('',(-34.,8.9,32.25));
#43387=CARTESIAN_POINT('',(-34.,8.9,31.4));
#43388=CARTESIAN_POINT('Origin',(-34.,9.,31.));
#43389=CARTESIAN_POINT('',(33.9,9.,31.1));
#43390=CARTESIAN_POINT('',(33.9,9.,32.25));
#43391=CARTESIAN_POINT('',(-34.,9.,31.1));
#43392=CARTESIAN_POINT('Origin',(33.95,8.95,32.25));
#43393=CARTESIAN_POINT('',(34.,8.9,31.4));
#43394=CARTESIAN_POINT('',(34.,8.9,31.4));
#43395=CARTESIAN_POINT('',(34.,8.9,31.1));
#43396=CARTESIAN_POINT('',(34.,8.9,32.25));
#43397=CARTESIAN_POINT('',(33.95,8.95,31.05));
#43398=CARTESIAN_POINT('',(34.,8.9,31.1));
#43399=CARTESIAN_POINT('',(22.4250000000009,20.4749999999997,42.5749999999999));
#43400=CARTESIAN_POINT('Origin',(-34.,8.95,31.05));
#43401=CARTESIAN_POINT('',(33.9,8.9,31.));
#43402=CARTESIAN_POINT('',(22.0083333333343,-2.99166666666635,19.1083333333334));
#43403=CARTESIAN_POINT('',(-33.9,8.9,31.));
#43404=CARTESIAN_POINT('',(-34.,8.9,31.));
#43405=CARTESIAN_POINT('',(-33.3416666666667,8.34166666666665,30.4416666666666));
#43406=CARTESIAN_POINT('Origin',(-34.,4.45,35.95));
#43407=CARTESIAN_POINT('',(33.95,4.45,35.95));
#43408=CARTESIAN_POINT('',(33.9,4.5,35.9));
#43409=CARTESIAN_POINT('',(22.0500000000009,16.3499999999997,24.0500000000001));
#43410=CARTESIAN_POINT('',(-33.9,4.5,35.9));
#43411=CARTESIAN_POINT('',(-34.,4.5,35.9));
#43412=CARTESIAN_POINT('',(-33.95,4.45,35.95));
#43413=CARTESIAN_POINT('',(-33.3833333333333,5.01666666666669,35.3833333333333));
#43414=CARTESIAN_POINT('',(-33.9,4.4,36.));
#43415=CARTESIAN_POINT('',(-34.1333333333333,4.63333333333334,35.7666666666667));
#43416=CARTESIAN_POINT('',(33.9,4.4,36.));
#43417=CARTESIAN_POINT('',(-34.,4.4,36.));
#43418=CARTESIAN_POINT('',(22.8000000000009,-6.69999999999966,47.0999999999999));
#43419=CARTESIAN_POINT('Origin',(-33.95,5.5,35.95));
#43420=CARTESIAN_POINT('',(-34.,4.4,35.9));
#43421=CARTESIAN_POINT('',(-34.,4.4,35.9));
#43422=CARTESIAN_POINT('',(-34.,4.1,35.9));
#43423=CARTESIAN_POINT('',(-34.,5.5,35.9));
#43424=CARTESIAN_POINT('',(-33.95,4.05,35.95));
#43425=CARTESIAN_POINT('',(-34.,4.1,35.9));
#43426=CARTESIAN_POINT('',(-33.9,4.1,36.));
#43427=CARTESIAN_POINT('',(-33.7166666666667,4.28333333333336,36.1833333333334));
#43428=CARTESIAN_POINT('',(-33.9,5.5,36.));
#43429=CARTESIAN_POINT('Origin',(-33.95,4.45,32.5));
#43430=CARTESIAN_POINT('',(-33.9,4.5,31.5));
#43431=CARTESIAN_POINT('',(-33.9,4.5,32.5));
#43432=CARTESIAN_POINT('',(-34.,4.4,31.4));
#43433=CARTESIAN_POINT('',(-34.,4.4,31.4));
#43434=CARTESIAN_POINT('',(-34.,4.4,32.5));
#43435=CARTESIAN_POINT('Origin',(-34.,4.5,31.5));
#43436=CARTESIAN_POINT('',(33.9,4.5,31.5));
#43437=CARTESIAN_POINT('',(33.9,4.5,32.5));
#43438=CARTESIAN_POINT('',(-34.,4.5,31.5));
#43439=CARTESIAN_POINT('',(29.025,4.5,33.5));
#43440=CARTESIAN_POINT('Origin',(30.,4.5,33.5));
#43441=CARTESIAN_POINT('',(-30.975,4.5,33.5));
#43442=CARTESIAN_POINT('Origin',(-30.,4.5,33.5));
#43443=CARTESIAN_POINT('Origin',(-34.,4.05,31.05));
#43444=CARTESIAN_POINT('',(33.95,4.05,31.05));
#43445=CARTESIAN_POINT('',(33.9,4.,31.1));
#43446=CARTESIAN_POINT('',(22.0083333333343,-7.89166666666636,42.9916666666666));
#43447=CARTESIAN_POINT('',(-33.9,4.,31.1));
#43448=CARTESIAN_POINT('',(-34.,4.,31.1));
#43449=CARTESIAN_POINT('',(-33.95,4.05,31.05));
#43450=CARTESIAN_POINT('',(-33.3416666666667,3.44166666666664,31.6583333333334));
#43451=CARTESIAN_POINT('',(-33.9,4.1,31.));
#43452=CARTESIAN_POINT('',(-33.7583333333333,4.24166666666667,30.8583333333333));
#43453=CARTESIAN_POINT('',(33.9,4.1,31.));
#43454=CARTESIAN_POINT('',(-34.,4.1,31.));
#43455=CARTESIAN_POINT('',(22.4250000000009,15.5749999999997,19.5250000000001));
#43456=CARTESIAN_POINT('Origin',(-33.95,4.05,34.75));
#43457=CARTESIAN_POINT('',(-33.9,4.,35.9));
#43458=CARTESIAN_POINT('',(-33.9,4.,34.75));
#43459=CARTESIAN_POINT('',(-33.7583333333333,3.85833333333333,35.7583333333333));
#43460=CARTESIAN_POINT('',(-34.,4.1,31.1));
#43461=CARTESIAN_POINT('',(-34.,4.1,34.75));
#43462=CARTESIAN_POINT('',(-34.,4.1,31.1));
#43463=CARTESIAN_POINT('Origin',(-34.,4.,36.));
#43464=CARTESIAN_POINT('',(33.9,4.,35.9));
#43465=CARTESIAN_POINT('',(33.9,4.,34.75));
#43466=CARTESIAN_POINT('',(-34.,4.,35.9));
#43467=CARTESIAN_POINT('',(-30.975,4.,33.5));
#43468=CARTESIAN_POINT('Origin',(-30.,4.,33.5));
#43469=CARTESIAN_POINT('',(29.025,4.,33.5));
#43470=CARTESIAN_POINT('Origin',(30.,4.,33.5));
#43471=CARTESIAN_POINT('Origin',(33.95,4.05,34.75));
#43472=CARTESIAN_POINT('',(34.,4.1,31.1));
#43473=CARTESIAN_POINT('',(34.,4.1,31.1));
#43474=CARTESIAN_POINT('',(34.,4.1,35.9));
#43475=CARTESIAN_POINT('',(34.,4.1,34.75));
#43476=CARTESIAN_POINT('',(33.95,4.05,35.95));
#43477=CARTESIAN_POINT('',(34.,4.1,35.9));
#43478=CARTESIAN_POINT('',(22.4250000000004,-7.4750000000002,24.4250000000004));
#43479=CARTESIAN_POINT('Origin',(-34.,4.05,35.95));
#43480=CARTESIAN_POINT('',(33.9,4.1,36.));
#43481=CARTESIAN_POINT('',(22.3833333333348,15.6166666666666,47.516666666666));
#43482=CARTESIAN_POINT('',(-34.,4.1,36.));
#43483=CARTESIAN_POINT('Origin',(33.95,5.5,35.95));
#43484=CARTESIAN_POINT('',(33.9,5.5,36.));
#43485=CARTESIAN_POINT('',(34.,4.4,35.9));
#43486=CARTESIAN_POINT('',(34.,5.5,35.9));
#43487=CARTESIAN_POINT('',(34.,4.4,35.9));
#43488=CARTESIAN_POINT('Origin',(30.,4.45,33.5));
#43489=CARTESIAN_POINT('',(29.125,4.4,33.5));
#43490=CARTESIAN_POINT('',(29.075,4.45,33.5));
#43491=CARTESIAN_POINT('Origin',(30.,4.4,33.5));
#43492=CARTESIAN_POINT('Origin',(30.,0.,33.5));
#43493=CARTESIAN_POINT('',(29.125,4.1,33.5));
#43494=CARTESIAN_POINT('Origin',(30.,4.1,33.5));
#43495=CARTESIAN_POINT('',(29.125,0.,33.5));
#43496=CARTESIAN_POINT('Origin',(30.,4.05,33.5));
#43497=CARTESIAN_POINT('',(29.075,4.05,33.5));
#43498=CARTESIAN_POINT('Origin',(-30.,4.45,33.5));
#43499=CARTESIAN_POINT('',(-30.875,4.4,33.5));
#43500=CARTESIAN_POINT('',(-30.925,4.45,33.5));
#43501=CARTESIAN_POINT('Origin',(-30.,4.4,33.5));
#43502=CARTESIAN_POINT('Origin',(-30.,0.,33.5));
#43503=CARTESIAN_POINT('',(-30.875,4.1,33.5));
#43504=CARTESIAN_POINT('Origin',(-30.,4.1,33.5));
#43505=CARTESIAN_POINT('',(-30.875,0.,33.5));
#43506=CARTESIAN_POINT('Origin',(-30.,4.05,33.5));
#43507=CARTESIAN_POINT('',(-30.925,4.05,33.5));
#43508=CARTESIAN_POINT('Origin',(33.95,4.45,32.5));
#43509=CARTESIAN_POINT('',(34.,4.4,31.4));
#43510=CARTESIAN_POINT('',(34.,4.4,32.5));
#43511=CARTESIAN_POINT('',(34.,4.4,31.4));
#43512=CARTESIAN_POINT('Origin',(33.95,7.75,31.45));
#43513=CARTESIAN_POINT('',(33.9,7.75,31.5));
#43514=CARTESIAN_POINT('',(34.,7.75,31.4));
#43515=CARTESIAN_POINT('Origin',(33.95,5.25,31.05));
#43516=CARTESIAN_POINT('',(34.,5.25,31.1));
#43517=CARTESIAN_POINT('',(33.9,5.25,31.));
#43518=CARTESIAN_POINT('Origin',(-34.,4.5,36.));
#43519=CARTESIAN_POINT('Origin',(34.,6.5,33.5));
#43520=CARTESIAN_POINT('Origin',(-33.95,5.25,31.05));
#43521=CARTESIAN_POINT('',(-33.9,5.25,31.));
#43522=CARTESIAN_POINT('',(-34.,5.25,31.1));
#43523=CARTESIAN_POINT('Origin',(-33.95,7.75,31.45));
#43524=CARTESIAN_POINT('',(-34.,7.75,31.4));
#43525=CARTESIAN_POINT('',(-33.9,7.75,31.5));
#43526=CARTESIAN_POINT('Origin',(-34.,4.,31.));
#43527=CARTESIAN_POINT('Origin',(-34.,6.5,33.5));
#43528=CARTESIAN_POINT('Origin',(-34.,9.,31.5));
#71455=UNCERTAINTY_MEASURE_WITH_UNIT(LENGTH_MEASURE(0.001),#71493,
'DISTANCE_ACCURACY_VALUE',
'Maximum model space distance between geometric entities at asserted c
onnectivities');
#71471=UNCERTAINTY_MEASURE_WITH_UNIT(LENGTH_MEASURE(0.001),#71493,
'DISTANCE_ACCURACY_VALUE',
'Maximum model space distance between geometric entities at asserted c
onnectivities');
#71476=(
GEOMETRIC_REPRESENTATION_CONTEXT(3)
GLOBAL_UNCERTAINTY_ASSIGNED_CONTEXT((#71455))
GLOBAL_UNIT_ASSIGNED_CONTEXT((#71493,#71495,#71496))
REPRESENTATION_CONTEXT('','3D')
);
#71492=(
GEOMETRIC_REPRESENTATION_CONTEXT(3)
GLOBAL_UNCERTAINTY_ASSIGNED_CONTEXT((#71471))
GLOBAL_UNIT_ASSIGNED_CONTEXT((#71493,#71495,#71496))
REPRESENTATION_CONTEXT('','3D')
);
#71493=(
LENGTH_UNIT()
NAMED_UNIT(*)
SI_UNIT(.CENTI.,.METRE.)
);
#71495=(
NAMED_UNIT(*)
PLANE_ANGLE_UNIT()
SI_UNIT($,.RADIAN.)
);
#71496=(
NAMED_UNIT(*)
SI_UNIT($,.STERADIAN.)
SOLID_ANGLE_UNIT()
);
#71501=SHAPE_DEFINITION_REPRESENTATION(#71521,#71606);
#71521=PRODUCT_DEFINITION_SHAPE('',$,#71627);
#71606=SHAPE_REPRESENTATION('',(#29306),#71476);
#71622=PRODUCT_DEFINITION_CONTEXT('part definition',#71684,'design');
#71627=PRODUCT_DEFINITION('2026-10-19-03-21-58-368',
'08_Lower_Cross_Brace_L680_L50x50x5',#71647,#71622);
#71647=PRODUCT_DEFINITION_FORMATION('',$,#71690);
#71684=APPLICATION_CONTEXT(
'Core Data for Automotive Mechanical Design Process');
#71685=PRODUCT_CONTEXT('part definition',#71684,'mechanical');
#71690=PRODUCT('2026-10-19-03-21-58-368',
'08_Lower_Cross_Brace_L680_L50x50x5',$,(#71685));
#71867=COLOUR_RGB('Light Blue',0.38,0.62,0.78);
#71868=FILL_AREA_STYLE_COLOUR('',#71867);
#71869=FILL_AREA_STYLE('',(#71868));
#71870=SURFACE_STYLE_FILL_AREA(#71869);
#71871=SURFACE_SIDE_STYLE('',(#71870));
#71872=SURFACE_STYLE_USAGE(.BOTH.,#71871);
#71873=PRESENTATION_STYLE_ASSIGNMENT((#71872));
ENDSEC;
END-ISO-10303-21;
